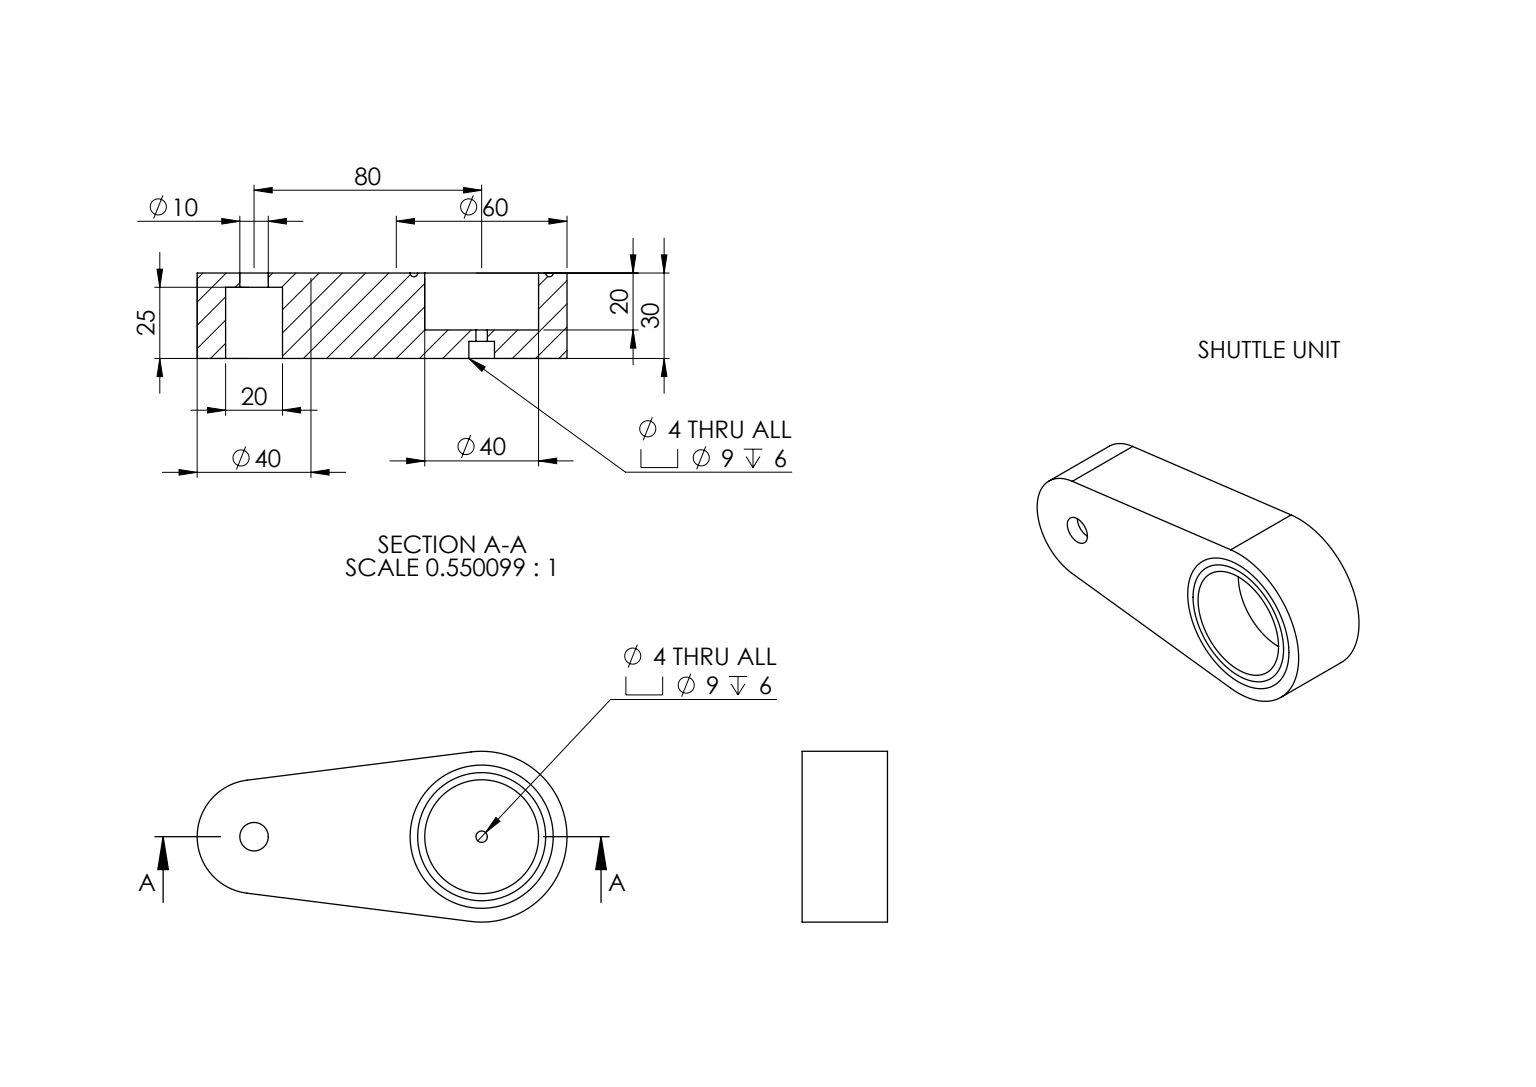
ISO-10303-21;
HEADER;
FILE_DESCRIPTION (('STEP AP214'),
    '1' );
FILE_NAME ('shuttle unit.step',
    '2026-10-24T08:20:21',
    ( '' ),
    ( '' ),
    'SwSTEP 2.0',
    'SolidWorks 2026',
    '' );
FILE_SCHEMA (( 'AUTOMOTIVE_DESIGN' ));
ENDSEC;

DATA;
#22=CARTESIAN_POINT ( 'NONE',  ( 0.000000000000000000, 0.000000000000000000, -30.00000000000000000 ) ) ;
#26=EDGE_CURVE ( 'NONE', #192, #3050, #3399, .T. ) ;
#35=CIRCLE ( 'NONE', #2208, 22.50000000000000355 ) ;
#36=ORIENTED_EDGE ( 'NONE', *, *, #1121, .F. ) ;
#52=VERTEX_POINT ( 'NONE', #3188 ) ;
#58=DIRECTION ( 'NONE',  ( 0.1250000000000000833, 0.9921567416492215186, -0.000000000000000000 ) ) ;
#59=DIRECTION ( 'NONE',  ( 1.000000000000000000, 0.000000000000000000, 0.000000000000000000 ) ) ;
#64=DIRECTION ( 'NONE',  ( -1.000000000000000000, 0.000000000000000000, 0.000000000000000000 ) ) ;
#70=DIRECTION ( 'NONE',  ( -1.000000000000000000, 0.000000000000000000, 0.000000000000000000 ) ) ;
#74=TOROIDAL_SURFACE ( 'NONE', #3494, 23.82500000000000284, 1.324999999999999956 ) ;
#77=DIRECTION ( 'NONE',  ( -1.000000000000000000, 0.000000000000000000, 0.000000000000000000 ) ) ;
#85=CARTESIAN_POINT ( 'NONE',  ( 0.000000000000000000, 0.000000000000000000, -30.00000000000000000 ) ) ;
#87=CARTESIAN_POINT ( 'NONE',  ( 0.000000000000000000, 0.000000000000000000, 0.000000000000000000 ) ) ;
#88=VECTOR ( 'NONE', #755, 999.9999999999998863 ) ;
#101=CARTESIAN_POINT ( 'NONE',  ( -85.00000000000000000, 0.000000000000000000, 0.001000000000000132727 ) ) ;
#103=CARTESIAN_POINT ( 'NONE',  ( -90.00000000000000000, 0.000000000000000000, -4.999999999999997335 ) ) ;
#107=CARTESIAN_POINT ( 'NONE',  ( -82.50000000000000000, -19.84313483298442904, 0.000000000000000000 ) ) ;
#115=ORIENTED_EDGE ( 'NONE', *, *, #3737, .T. ) ;
#116=PLANE ( 'NONE',  #1634 ) ;
#128=CARTESIAN_POINT ( 'NONE',  ( -80.00000000000000000, 0.000000000000000000, -30.00000000000000000 ) ) ;
#141=VECTOR ( 'NONE', #617, 1000.000000000000000 ) ;
#142=FACE_OUTER_BOUND ( 'NONE', #2988, .T. ) ;
#143=VERTEX_POINT ( 'NONE', #2588 ) ;
#159=SHAPE_REPRESENTATION ( 'shuttle unit', ( #2207 ), #968 ) ;
#161=EDGE_LOOP ( 'NONE', ( #2165, #1220, #1169, #2717, #1654 ) ) ;
#162=EDGE_CURVE ( 'NONE', #3091, #1782, #1381, .T. ) ;
#164=EDGE_CURVE ( 'NONE', #494, #1780, #3780, .T. ) ;
#166=CARTESIAN_POINT ( 'NONE',  ( 20.00000000000000000, 0.000000000000000000, 0.000000000000000000 ) ) ;
#178=ORIENTED_EDGE ( 'NONE', *, *, #1295, .F. ) ;
#179=CARTESIAN_POINT ( 'NONE',  ( -80.00000000000000000, 0.000000000000000000, 0.001000000000000132727 ) ) ;
#180=ORIENTED_EDGE ( 'NONE', *, *, #2925, .T. ) ;
#186=ORIENTED_EDGE ( 'NONE', *, *, #1295, .T. ) ;
#190=DIRECTION ( 'NONE',  ( -0.000000000000000000, 0.000000000000000000, 1.000000000000000000 ) ) ;
#192=VERTEX_POINT ( 'NONE', #3809 ) ;
#207=AXIS2_PLACEMENT_3D ( 'NONE', #2463, #2835, #972 ) ;
#215=CIRCLE ( 'NONE', #1581, 4.500000000000000888 ) ;
#223=ORIENTED_EDGE ( 'NONE', *, *, #2872, .T. ) ;
#233=SURFACE_SIDE_STYLE ('',( #1990 ) ) ;
#242=EDGE_LOOP ( 'NONE', ( #1908, #2671, #1653, #2183 ) ) ;
#255=DIRECTION ( 'NONE',  ( 0.000000000000000000, 0.000000000000000000, 1.000000000000000000 ) ) ;
#256=CYLINDRICAL_SURFACE ( 'NONE', #2880, 20.00000000000000000 ) ;
#261=VERTEX_POINT ( 'NONE', #657 ) ;
#273=AXIS2_PLACEMENT_3D ( 'NONE', #2448, #3041, #3118 ) ;
#276=VERTEX_POINT ( 'NONE', #1202 ) ;
#285=DIRECTION ( 'NONE',  ( -1.000000000000000000, 0.000000000000000000, 0.000000000000000000 ) ) ;
#296=CARTESIAN_POINT ( 'NONE',  ( 23.18826319173439288, -9.737913028511604452, 0.000000000000000000 ) ) ;
#301=ORIENTED_EDGE ( 'NONE', *, *, #2925, .F. ) ;
#302=FACE_OUTER_BOUND ( 'NONE', #2329, .T. ) ;
#304=EDGE_CURVE ( 'NONE', #2072, #2934, #2995, .T. ) ;
#307=ORIENTED_EDGE ( 'NONE', *, *, #1137, .F. ) ;
#321=CARTESIAN_POINT ( 'NONE',  ( 0.000000000000000000, 0.000000000000000000, -30.00000000000000000 ) ) ;
#326=ORIENTED_EDGE ( 'NONE', *, *, #2063, .T. ) ;
#328=VERTEX_POINT ( 'NONE', #1471 ) ;
#332=AXIS2_PLACEMENT_3D ( 'NONE', #2007, #2609, #441 ) ;
#346=PLANE ( 'NONE',  #504 ) ;
#349=CARTESIAN_POINT ( 'NONE',  ( 0.000000000000000000, 0.000000000000000000, -30.00000000000000000 ) ) ;
#355=VERTEX_POINT ( 'NONE', #1451 ) ;
#361=ADVANCED_FACE ( 'NONE', ( #2704, #2412, #2101 ), #1506, .T. ) ;
#363=DIRECTION ( 'NONE',  ( -1.000000000000000000, 0.000000000000000000, 0.000000000000000000 ) ) ;
#369=DIRECTION ( 'NONE',  ( -1.000000000000000000, 0.000000000000000000, 0.000000000000000000 ) ) ;
#372=DIRECTION ( 'NONE',  ( -0.9921567416492215186, 0.1250000000000000833, 0.000000000000000000 ) ) ;
#375=CARTESIAN_POINT ( 'NONE',  ( 0.000000000000000000, 0.000000000000000000, -30.00000000000000000 ) ) ;
#377=CIRCLE ( 'NONE', #827, 5.000000000000004441 ) ;
#379=CIRCLE ( 'NONE', #1823, 9.999999999999994671 ) ;
#381=DIRECTION ( 'NONE',  ( -0.000000000000000000, 0.000000000000000000, 1.000000000000000000 ) ) ;
#385=VERTEX_POINT ( 'NONE', #3241 ) ;
#389=ADVANCED_FACE ( 'NONE', ( #2979, #1826 ), #580, .T. ) ;
#390=CARTESIAN_POINT ( 'NONE',  ( 0.000000000000000000, 0.000000000000000000, -20.00000000000000000 ) ) ;
#394=DIRECTION ( 'NONE',  ( -0.3871933609746165406, -0.9219985364506716463, 2.410490433790582225E-18 ) ) ;
#397=VECTOR ( 'NONE', #716, 1000.000000000000000 ) ;
#406=ORIENTED_EDGE ( 'NONE', *, *, #3273, .T. ) ;
#411=ORIENTED_EDGE ( 'NONE', *, *, #905, .T. ) ;
#425=FACE_OUTER_BOUND ( 'NONE', #911, .T. ) ;
#434=DIRECTION ( 'NONE',  ( -0.000000000000000000, -0.000000000000000000, 1.000000000000000000 ) ) ;
#441=DIRECTION ( 'NONE',  ( 1.000000000000000000, 0.000000000000000000, 0.000000000000000000 ) ) ;
#443=AXIS2_PLACEMENT_3D ( 'NONE', #885, #2071, #3254 ) ;
#446=FACE_OUTER_BOUND ( 'NONE', #1984, .T. ) ;
#452=DIRECTION ( 'NONE',  ( -1.000000000000000000, 0.000000000000000000, 0.000000000000000000 ) ) ;
#454=FACE_OUTER_BOUND ( 'NONE', #746, .T. ) ;
#464=UNCERTAINTY_MEASURE_WITH_UNIT (LENGTH_MEASURE( 1.000000000000000082E-05 ), #2003, 'distance_accuracy_value', 'NONE');
#493=DIRECTION ( 'NONE',  ( 1.000000000000000000, 0.000000000000000000, 0.000000000000000000 ) ) ;
#494=VERTEX_POINT ( 'NONE', #975 ) ;
#495=DIRECTION ( 'NONE',  ( -0.000000000000000000, -0.000000000000000000, -1.000000000000000000 ) ) ;
#501=CARTESIAN_POINT ( 'NONE',  ( 0.000000000000000000, -0.000000000000000000, 0.000000000000000000 ) ) ;
#504=AXIS2_PLACEMENT_3D ( 'NONE', #2399, #1248, #996 ) ;
#515=DIRECTION ( 'NONE',  ( 0.000000000000000000, -1.000000000000000000, 0.000000000000000000 ) ) ;
#516=EDGE_CURVE ( 'NONE', #3615, #1351, #3346, .T. ) ;
#517=EDGE_CURVE ( 'NONE', #1737, #494, #1548, .T. ) ;
#528=AXIS2_PLACEMENT_3D ( 'NONE', #2164, #3336, #2490 ) ;
#530=DIRECTION ( 'NONE',  ( -1.000000000000000000, 0.000000000000000000, -0.000000000000000000 ) ) ;
#531=EDGE_LOOP ( 'NONE', ( #830, #1241, #942, #1732 ) ) ;
#540=DIRECTION ( 'NONE',  ( -0.000000000000000000, -0.000000000000000000, -1.000000000000000000 ) ) ;
#546=EDGE_CURVE ( 'NONE', #671, #2369, #590, .T. ) ;
#550=ORIENTED_EDGE ( 'NONE', *, *, #2872, .F. ) ;
#553=DIRECTION ( 'NONE',  ( 0.000000000000000000, -1.000000000000000000, 0.000000000000000000 ) ) ;
#563=EDGE_LOOP ( 'NONE', ( #2991, #2903, #3738, #178 ) ) ;
#566=EDGE_CURVE ( 'NONE', #3824, #3666, #844, .T. ) ;
#573=VERTEX_POINT ( 'NONE', #1808 ) ;
#575=FACE_BOUND ( 'NONE', #2885, .T. ) ;
#576=( GEOMETRIC_REPRESENTATION_CONTEXT ( 3 ) GLOBAL_UNCERTAINTY_ASSIGNED_CONTEXT ( ( #464 ) ) GLOBAL_UNIT_ASSIGNED_CONTEXT ( ( #2003, #2025, #3522 ) ) REPRESENTATION_CONTEXT ( 'NONE', 'WORKASPACE' ) );
#580=PLANE ( 'NONE',  #2653 ) ;
#581=CARTESIAN_POINT ( 'NONE',  ( 0.000000000000000000, -0.000000000000000000, 0.000000000000000000 ) ) ;
#590=CIRCLE ( 'NONE', #2764, 1.325000000000000622 ) ;
#593=CIRCLE ( 'NONE', #2088, 4.500000000000000888 ) ;
#595=CARTESIAN_POINT ( 'NONE',  ( -80.00000000000000000, 0.000000000000000000, -4.999999999999997335 ) ) ;
#598=AXIS2_PLACEMENT_3D ( 'NONE', #3513, #255, #2913 ) ;
#610=ORIENTED_EDGE ( 'NONE', *, *, #809, .F. ) ;
#617=DIRECTION ( 'NONE',  ( -0.000000000000000000, -0.000000000000000000, -1.000000000000000000 ) ) ;
#622=FACE_OUTER_BOUND ( 'NONE', #2781, .T. ) ;
#630=ORIENTED_EDGE ( 'NONE', *, *, #750, .T. ) ;
#641=DIRECTION ( 'NONE',  ( -0.9921567416492214075, 0.1250000000000000555, 0.000000000000000000 ) ) ;
#652=DIRECTION ( 'NONE',  ( 1.000000000000000000, 0.000000000000000000, 0.000000000000000000 ) ) ;
#655=EDGE_LOOP ( 'NONE', ( #3357, #2286, #1960, #1641, #907, #1356, #3483, #1912 ) ) ;
#657=CARTESIAN_POINT ( 'NONE',  ( -90.00000000000000000, 0.000000000000000000, -30.00000000000000000 ) ) ;
#662=CARTESIAN_POINT ( 'NONE',  ( -80.00000000000000000, 0.000000000000000000, -30.00000000000000000 ) ) ;
#665=EDGE_CURVE ( 'NONE', #3091, #3418, #215, .T. ) ;
#668=DIRECTION ( 'NONE',  ( -0.000000000000000000, -0.000000000000000000, -1.000000000000000000 ) ) ;
#671=VERTEX_POINT ( 'NONE', #3621 ) ;
#675=CARTESIAN_POINT ( 'NONE',  ( -3.750000000000001776, -29.76470224947664178, -30.00000000000000000 ) ) ;
#678=ADVANCED_FACE ( 'NONE', ( #302 ), #2688, .F. ) ;
#696=AXIS2_PLACEMENT_3D ( 'NONE', #375, #3331, #59 ) ;
#697=CARTESIAN_POINT ( 'NONE',  ( 0.000000000000000000, 0.000000000000000000, 0.000000000000000000 ) ) ;
#699=DIRECTION ( 'NONE',  ( 1.000000000000000000, 0.000000000000000000, 0.000000000000000000 ) ) ;
#707=EDGE_CURVE ( 'NONE', #1234, #1780, #2652, .T. ) ;
#716=DIRECTION ( 'NONE',  ( -0.000000000000000000, -1.000000000000000000, -0.000000000000000000 ) ) ;
#724=DIRECTION ( 'NONE',  ( 1.000000000000000000, 0.000000000000000000, 0.000000000000000000 ) ) ;
#731=CARTESIAN_POINT ( 'NONE',  ( 0.000000000000000000, 0.000000000000000000, 0.000000000000000000 ) ) ;
#732=ORIENTED_EDGE ( 'NONE', *, *, #3728, .T. ) ;
#740=EDGE_CURVE ( 'NONE', #1954, #1234, #2219, .T. ) ;
#746=EDGE_LOOP ( 'NONE', ( #610, #2576 ) ) ;
#750=EDGE_CURVE ( 'NONE', #2723, #2369, #1277, .T. ) ;
#755=DIRECTION ( 'NONE',  ( 0.9921567416492215186, 0.1250000000000001665, 0.000000000000000000 ) ) ;
#757=VERTEX_POINT ( 'NONE', #1550 ) ;
#758=VERTEX_POINT ( 'NONE', #107 ) ;
#764=AXIS2_PLACEMENT_3D ( 'NONE', #179, #3725, #2829 ) ;
#769=PLANE ( 'NONE',  #2386 ) ;
#791=ADVANCED_BREP_SHAPE_REPRESENTATION ( '', ( #1966, #2207 ), #968 ) ;
#792=DIRECTION ( 'NONE',  ( 0.000000000000000000, 0.000000000000000000, 1.000000000000000000 ) ) ;
#803=DIRECTION ( 'NONE',  ( 1.000000000000000000, 0.000000000000000000, 0.000000000000000000 ) ) ;
#809=EDGE_CURVE ( 'NONE', #385, #671, #35, .T. ) ;
#813=CYLINDRICAL_SURFACE ( 'NONE', #1460, 4.499999999999997335 ) ;
#820=CARTESIAN_POINT ( 'NONE',  ( 0.000000000000000000, 0.000000000000000000, 0.000000000000000000 ) ) ;
#826=CIRCLE ( 'NONE', #1320, 20.00000000000000355 ) ;
#827=AXIS2_PLACEMENT_3D ( 'NONE', #1745, #2304, #2589 ) ;
#830=ORIENTED_EDGE ( 'NONE', *, *, #809, .T. ) ;
#838=CARTESIAN_POINT ( 'NONE',  ( 0.000000000000000000, 0.000000000000000000, -30.00000000000000000 ) ) ;
#844=CIRCLE ( 'NONE', #3019, 30.00000000000000000 ) ;
#849=CYLINDRICAL_SURFACE ( 'NONE', #764, 5.000000000000004441 ) ;
#850=ORIENTED_EDGE ( 'NONE', *, *, #2359, .T. ) ;
#852=ORIENTED_EDGE ( 'NONE', *, *, #1811, .T. ) ;
#853=PRODUCT_DEFINITION_FORMATION_WITH_SPECIFIED_SOURCE ( 'ANY', '', #3643, .NOT_KNOWN. ) ;
#854=EDGE_CURVE ( 'NONE', #3666, #1351, #1907, .T. ) ;
#858=LINE ( 'NONE', #2300, #1159 ) ;
#862=ORIENTED_EDGE ( 'NONE', *, *, #1617, .F. ) ;
#885=CARTESIAN_POINT ( 'NONE',  ( 0.000000000000000000, 0.000000000000000000, 0.000000000000000000 ) ) ;
#887=CIRCLE ( 'NONE', #2621, 5.000000000000004441 ) ;
#891=CARTESIAN_POINT ( 'NONE',  ( 0.000000000000000000, 0.000000000000000000, -30.00000000000000000 ) ) ;
#894=AXIS2_PLACEMENT_3D ( 'NONE', #2296, #1423, #1955 ) ;
#900=VECTOR ( 'NONE', #3282, 1000.000000000000000 ) ;
#905=EDGE_CURVE ( 'NONE', #1737, #2422, #2837, .T. ) ;
#907=ORIENTED_EDGE ( 'NONE', *, *, #566, .F. ) ;
#911=EDGE_LOOP ( 'NONE', ( #1275, #2494 ) ) ;
#914=LINE ( 'NONE', #2097, #900 ) ;
#918=CARTESIAN_POINT ( 'NONE',  ( 20.00000000000000000, 0.000000000000000000, -20.00000000000000000 ) ) ;
#927=ORIENTED_EDGE ( 'NONE', *, *, #3644, .T. ) ;
#937=ADVANCED_FACE ( 'NONE', ( #3402, #454 ), #2465, .T. ) ;
#938=DIRECTION ( 'NONE',  ( 1.000000000000000000, 0.000000000000000000, 0.000000000000000000 ) ) ;
#942=ORIENTED_EDGE ( 'NONE', *, *, #3532, .T. ) ;
#943=EDGE_CURVE ( 'NONE', #1799, #2993, #2254, .T. ) ;
#945=LINE ( 'NONE', #2951, #1884 ) ;
#952=AXIS2_PLACEMENT_3D ( 'NONE', #2980, #2082, #70 ) ;
#962=DIRECTION ( 'NONE',  ( 0.000000000000000000, 0.000000000000000000, 1.000000000000000000 ) ) ;
#963=DIRECTION ( 'NONE',  ( -1.000000000000000000, 0.000000000000000000, 0.000000000000000000 ) ) ;
#968=( GEOMETRIC_REPRESENTATION_CONTEXT ( 3 ) GLOBAL_UNCERTAINTY_ASSIGNED_CONTEXT ( ( #3201 ) ) GLOBAL_UNIT_ASSIGNED_CONTEXT ( ( #2883, #3143, #1928 ) ) REPRESENTATION_CONTEXT ( 'NONE', 'WORKASPACE' ) );
#971=VECTOR ( 'NONE', #1427, 1000.000000000000114 ) ;
#972=DIRECTION ( 'NONE',  ( -1.000000000000000000, 0.000000000000000000, 0.000000000000000000 ) ) ;
#975=CARTESIAN_POINT ( 'NONE',  ( -70.00000000000000000, -21.41798680385620202, -30.00000000000000000 ) ) ;
#977=EDGE_CURVE ( 'NONE', #3418, #3091, #593, .T. ) ;
#991=DIRECTION ( 'NONE',  ( -0.000000000000000000, -0.000000000000000000, -1.000000000000000000 ) ) ;
#996=DIRECTION ( 'NONE',  ( -0.000000000000000000, 0.000000000000000000, 1.000000000000000000 ) ) ;
#999=DIRECTION ( 'NONE',  ( -0.000000000000000000, -0.000000000000000000, -1.000000000000000000 ) ) ;
#1003=VERTEX_POINT ( 'NONE', #3667 ) ;
#1008=CARTESIAN_POINT ( 'NONE',  ( -3.750000000000001776, -29.76470224947664178, -4.999999999999997335 ) ) ;
#1009=EDGE_CURVE ( 'NONE', #1780, #573, #3113, .T. ) ;
#1014=ORIENTED_EDGE ( 'NONE', *, *, #665, .F. ) ;
#1021=DIRECTION ( 'NONE',  ( 0.3871933609746164295, 0.9219985364506716463, -2.410490433790583766E-18 ) ) ;
#1024=EDGE_LOOP ( 'NONE', ( #862, #732, #2751, #550 ) ) ;
#1031=DIRECTION ( 'NONE',  ( -1.000000000000000000, 0.000000000000000000, 0.000000000000000000 ) ) ;
#1037=DIRECTION ( 'NONE',  ( 1.000000000000000000, 0.000000000000000000, 0.000000000000000000 ) ) ;
#1063=ORIENTED_EDGE ( 'NONE', *, *, #164, .T. ) ;
#1068=VERTEX_POINT ( 'NONE', #2932 ) ;
#1077=AXIS2_PLACEMENT_3D ( 'NONE', #128, #1951, #1325 ) ;
#1080=AXIS2_PLACEMENT_3D ( 'NONE', #3179, #530, #2863 ) ;
#1090=FACE_OUTER_BOUND ( 'NONE', #2921, .T. ) ;
#1094=EDGE_LOOP ( 'NONE', ( #1195, #2367 ) ) ;
#1101=CIRCLE ( 'NONE', #1965, 2.000000000000001776 ) ;
#1102=CARTESIAN_POINT ( 'NONE',  ( 0.000000000000000000, 0.000000000000000000, 0.000000000000000000 ) ) ;
#1109=ORIENTED_EDGE ( 'NONE', *, *, #1617, .T. ) ;
#1111=CARTESIAN_POINT ( 'NONE',  ( 2.000000000000001776, 0.000000000000000000, -24.00000000000000000 ) ) ;
#1114=DIRECTION ( 'NONE',  ( 0.000000000000000000, 0.000000000000000000, 1.000000000000000000 ) ) ;
#1120=EDGE_LOOP ( 'NONE', ( #2830, #326, #2091, #1837 ) ) ;
#1121=EDGE_CURVE ( 'NONE', #1151, #3615, #1672, .T. ) ;
#1124=CARTESIAN_POINT ( 'NONE',  ( -82.50000000000000000, 19.84313483298442193, -30.00000000000000000 ) ) ;
#1125=DIRECTION ( 'NONE',  ( -1.000000000000000000, 0.000000000000000000, 0.000000000000000000 ) ) ;
#1126=EDGE_CURVE ( 'NONE', #355, #2934, #3519, .T. ) ;
#1127=ORIENTED_EDGE ( 'NONE', *, *, #1126, .F. ) ;
#1133=EDGE_CURVE ( 'NONE', #1954, #494, #858, .T. ) ;
#1137=EDGE_CURVE ( 'NONE', #143, #1068, #1101, .T. ) ;
#1140=ADVANCED_FACE ( 'NONE', ( #1090 ), #813, .F. ) ;
#1151=VERTEX_POINT ( 'NONE', #3205 ) ;
#1159=VECTOR ( 'NONE', #553, 1000.000000000000000 ) ;
#1160=ORIENTED_EDGE ( 'NONE', *, *, #3532, .F. ) ;
#1169=ORIENTED_EDGE ( 'NONE', *, *, #707, .T. ) ;
#1174=ORIENTED_EDGE ( 'NONE', *, *, #3728, .F. ) ;
#1185=CARTESIAN_POINT ( 'NONE',  ( -80.00000000000000000, 0.000000000000000000, -4.999999999999997335 ) ) ;
#1192=TOROIDAL_SURFACE ( 'NONE', #1316, 23.82500000000000284, 1.324999999999999956 ) ;
#1194=DIRECTION ( 'NONE',  ( -0.000000000000000000, -0.000000000000000000, 1.000000000000000000 ) ) ;
#1195=ORIENTED_EDGE ( 'NONE', *, *, #1897, .F. ) ;
#1199=AXIS2_PLACEMENT_3D ( 'NONE', #1111, #2352, #2642 ) ;
#1202=CARTESIAN_POINT ( 'NONE',  ( -90.00000000000000000, -17.32050807568877815, -30.00000000000000000 ) ) ;
#1213=EDGE_CURVE ( 'NONE', #573, #758, #3350, .T. ) ;
#1217=AXIS2_PLACEMENT_3D ( 'NONE', #349, #2733, #963 ) ;
#1220=ORIENTED_EDGE ( 'NONE', *, *, #2326, .F. ) ;
#1233=DIRECTION ( 'NONE',  ( 1.000000000000000000, 0.000000000000000000, 0.000000000000000000 ) ) ;
#1234=VERTEX_POINT ( 'NONE', #1537 ) ;
#1241=ORIENTED_EDGE ( 'NONE', *, *, #546, .T. ) ;
#1248=DIRECTION ( 'NONE',  ( -1.000000000000000000, 0.000000000000000000, -0.000000000000000000 ) ) ;
#1275=ORIENTED_EDGE ( 'NONE', *, *, #3443, .T. ) ;
#1277=CIRCLE ( 'NONE', #273, 25.15000000000000213 ) ;
#1282=CARTESIAN_POINT ( 'NONE',  ( -3.749999999999998224, -29.76470224947664533, -30.00000000000000000 ) ) ;
#1284=EDGE_CURVE ( 'NONE', #261, #1954, #1523, .T. ) ;
#1286=CARTESIAN_POINT ( 'NONE',  ( -70.00000000000000000, 0.000000000000000000, -4.999999999999997335 ) ) ;
#1289=CARTESIAN_POINT ( 'NONE',  ( 0.000000000000000000, 0.000000000000000000, -30.00000000000000000 ) ) ;
#1295=EDGE_CURVE ( 'NONE', #2309, #1351, #2897, .T. ) ;
#1298=CARTESIAN_POINT ( 'NONE',  ( 0.000000000000000000, 0.000000000000000000, -24.00000000000000000 ) ) ;
#1310=LINE ( 'NONE', #2206, #1706 ) ;
#1311=LINE ( 'NONE', #101, #2818 ) ;
#1316=AXIS2_PLACEMENT_3D ( 'NONE', #501, #3743, #2848 ) ;
#1317=DIRECTION ( 'NONE',  ( 0.000000000000000000, 0.000000000000000000, 1.000000000000000000 ) ) ;
#1320=AXIS2_PLACEMENT_3D ( 'NONE', #595, #1194, #3572 ) ;
#1323=CIRCLE ( 'NONE', #1633, 4.499999999999993783 ) ;
#1325=DIRECTION ( 'NONE',  ( 1.000000000000000000, 0.000000000000000000, 0.000000000000000000 ) ) ;
#1331=DIRECTION ( 'NONE',  ( -0.9921567416492215186, 0.1250000000000000833, 0.000000000000000000 ) ) ;
#1332=FACE_OUTER_BOUND ( 'NONE', #2931, .T. ) ;
#1336=VECTOR ( 'NONE', #999, 1000.000000000000000 ) ;
#1342=CARTESIAN_POINT ( 'NONE',  ( 0.000000000000000000, 0.000000000000000000, -20.00000000000000000 ) ) ;
#1351=VERTEX_POINT ( 'NONE', #2801 ) ;
#1352=LINE ( 'NONE', #1992, #2194 ) ;
#1354=CARTESIAN_POINT ( 'NONE',  ( -3.750000000000004441, 29.76470224947664533, -30.00000000000000000 ) ) ;
#1356=ORIENTED_EDGE ( 'NONE', *, *, #2359, .F. ) ;
#1363=LINE ( 'NONE', #1608, #3303 ) ;
#1365=CYLINDRICAL_SURFACE ( 'NONE', #1077, 20.00000000000000355 ) ;
#1375=APPLICATION_CONTEXT ( 'automotive_design' ) ;
#1377=DIRECTION ( 'NONE',  ( -0.000000000000000000, -0.000000000000000000, 1.000000000000000000 ) ) ;
#1380=EDGE_LOOP ( 'NONE', ( #3293, #2842 ) ) ;
#1381=LINE ( 'NONE', #1715, #1407 ) ;
#1398=ORIENTED_EDGE ( 'NONE', *, *, #2612, .T. ) ;
#1406=ADVANCED_FACE ( 'NONE', ( #2861 ), #1192, .F. ) ;
#1407=VECTOR ( 'NONE', #540, 1000.000000000000000 ) ;
#1412=ORIENTED_EDGE ( 'NONE', *, *, #1811, .F. ) ;
#1423=DIRECTION ( 'NONE',  ( -0.000000000000000000, 0.000000000000000000, 1.000000000000000000 ) ) ;
#1427=DIRECTION ( 'NONE',  ( -0.9921567416492214075, 0.1250000000000000555, 0.000000000000000000 ) ) ;
#1428=CARTESIAN_POINT ( 'NONE',  ( -80.00000000000000000, 0.000000000000000000, -4.999999999999997335 ) ) ;
#1431=DIRECTION ( 'NONE',  ( -1.795453617517838654E-17, 1.015442787603507153E-17, 1.000000000000000000 ) ) ;
#1436=ADVANCED_FACE ( 'NONE', ( #3107 ), #1365, .T. ) ;
#1441=AXIS2_PLACEMENT_3D ( 'NONE', #891, #2663, #652 ) ;
#1445=DIRECTION ( 'NONE',  ( -0.000000000000000000, -0.000000000000000000, -1.000000000000000000 ) ) ;
#1447=CARTESIAN_POINT ( 'NONE',  ( -90.00000000000000000, 0.000000000000000000, -30.00000000000000000 ) ) ;
#1451=CARTESIAN_POINT ( 'NONE',  ( -20.00000000000000000, 2.449293598294706513E-15, 0.000000000000000000 ) ) ;
#1460=AXIS2_PLACEMENT_3D ( 'NONE', #1741, #1445, #2314 ) ;
#1462=ORIENTED_EDGE ( 'NONE', *, *, #750, .F. ) ;
#1467=CARTESIAN_POINT ( 'NONE',  ( -80.00000000000000000, 0.000000000000000000, -30.00000000000000000 ) ) ;
#1469=ORIENTED_EDGE ( 'NONE', *, *, #516, .T. ) ;
#1471=CARTESIAN_POINT ( 'NONE',  ( -20.00000000000000000, 2.449293598294706513E-15, -20.00000000000000000 ) ) ;
#1490=ORIENTED_EDGE ( 'NONE', *, *, #3224, .T. ) ;
#1491=DIRECTION ( 'NONE',  ( -1.000000000000000000, 0.000000000000000000, 0.000000000000000000 ) ) ;
#1496=AXIS2_PLACEMENT_3D ( 'NONE', #321, #1969, #724 ) ;
#1506=PLANE ( 'NONE',  #3764 ) ;
#1523=CIRCLE ( 'NONE', #1899, 9.999999999999994671 ) ;
#1534=PLANE ( 'NONE',  #696 ) ;
#1537=CARTESIAN_POINT ( 'NONE',  ( -70.00000000000000000, 0.000000000000000000, -4.999999999999997335 ) ) ;
#1548=LINE ( 'NONE', #675, #2274 ) ;
#1550=CARTESIAN_POINT ( 'NONE',  ( -85.00000000000000000, 0.000000000000000000, -4.999999999999997335 ) ) ;
#1557=ORIENTED_EDGE ( 'NONE', *, *, #740, .T. ) ;
#1558=DIRECTION ( 'NONE',  ( 0.1250000000000001665, -0.9921567416492215186, 0.000000000000000000 ) ) ;
#1562=DIRECTION ( 'NONE',  ( -0.000000000000000000, 0.000000000000000000, 1.000000000000000000 ) ) ;
#1564=STYLED_ITEM('',(#3860),#1966);
#1581=AXIS2_PLACEMENT_3D ( 'NONE', #2728, #2672, #1491 ) ;
#1591=DIRECTION ( 'NONE',  ( 0.000000000000000000, -0.000000000000000000, -1.000000000000000000 ) ) ;
#1595=FACE_OUTER_BOUND ( 'NONE', #1801, .T. ) ;
#1603=CARTESIAN_POINT ( 'NONE',  ( -3.750000000000004441, 29.76470224947664533, 0.000000000000000000 ) ) ;
#1608=CARTESIAN_POINT ( 'NONE',  ( -20.00000000000000000, 2.449293598294706513E-15, -20.00000000000000000 ) ) ;
#1617=EDGE_CURVE ( 'NONE', #1003, #2788, #3746, .T. ) ;
#1621=ORIENTED_EDGE ( 'NONE', *, *, #2989, .T. ) ;
#1633=AXIS2_PLACEMENT_3D ( 'NONE', #1289, #668, #77 ) ;
#1634=AXIS2_PLACEMENT_3D ( 'NONE', #1354, #1558, #1891 ) ;
#1641=ORIENTED_EDGE ( 'NONE', *, *, #1820, .T. ) ;
#1644=DIRECTION ( 'NONE',  ( -0.000000000000000000, -0.000000000000000000, -1.000000000000000000 ) ) ;
#1653=ORIENTED_EDGE ( 'NONE', *, *, #2499, .T. ) ;
#1654=ORIENTED_EDGE ( 'NONE', *, *, #3224, .F. ) ;
#1663=ADVANCED_FACE ( 'NONE', ( #2470, #3656 ), #1534, .F. ) ;
#1667=ADVANCED_FACE ( 'NONE', ( #3289 ), #346, .F. ) ;
#1672=LINE ( 'NONE', #1124, #2834 ) ;
#1675=CARTESIAN_POINT ( 'NONE',  ( -70.00000000000000000, -21.41798680385620202, -30.00000000000000000 ) ) ;
#1682=PLANE ( 'NONE',  #1080 ) ;
#1686=CARTESIAN_POINT ( 'NONE',  ( 4.500000000000000000, 5.510910596163089556E-16, -24.00000000000000000 ) ) ;
#1687=EDGE_LOOP ( 'NONE', ( #2677, #3663 ) ) ;
#1691=ORIENTED_EDGE ( 'NONE', *, *, #740, .F. ) ;
#1693=FACE_OUTER_BOUND ( 'NONE', #2600, .T. ) ;
#1697=FILL_AREA_STYLE ('',( #1952 ) ) ;
#1700=AXIS2_PLACEMENT_3D ( 'NONE', #3794, #3175, #1731 ) ;
#1706=VECTOR ( 'NONE', #1331, 999.9999999999998863 ) ;
#1711=FACE_OUTER_BOUND ( 'NONE', #1380, .T. ) ;
#1712=EDGE_CURVE ( 'NONE', #1151, #276, #3431, .T. ) ;
#1715=CARTESIAN_POINT ( 'NONE',  ( 4.499999999999997335, 5.510910596163085611E-16, -30.00000000000000000 ) ) ;
#1716=AXIS2_PLACEMENT_3D ( 'NONE', #2513, #381, #2144 ) ;
#1726=ORIENTED_EDGE ( 'NONE', *, *, #2799, .F. ) ;
#1731=DIRECTION ( 'NONE',  ( 1.000000000000000000, 0.000000000000000000, 0.000000000000000000 ) ) ;
#1732=ORIENTED_EDGE ( 'NONE', *, *, #3644, .F. ) ;
#1736=DIRECTION ( 'NONE',  ( -0.000000000000000000, -0.000000000000000000, -1.000000000000000000 ) ) ;
#1737=VERTEX_POINT ( 'NONE', #3043 ) ;
#1741=CARTESIAN_POINT ( 'NONE',  ( 0.000000000000000000, 0.000000000000000000, -30.00000000000000000 ) ) ;
#1743=ORIENTED_EDGE ( 'NONE', *, *, #2063, .F. ) ;
#1745=CARTESIAN_POINT ( 'NONE',  ( -80.00000000000000000, 0.000000000000000000, -4.999999999999997335 ) ) ;
#1746=ADVANCED_FACE ( 'NONE', ( #622 ), #3001, .T. ) ;
#1747=ORIENTED_EDGE ( 'NONE', *, *, #1712, .T. ) ;
#1750=SHAPE_REPRESENTATION_RELATIONSHIP ( 'NONE' , 'NONE' ,  #159, #791 ) ;
#1752=AXIS2_PLACEMENT_3D ( 'NONE', #662, #2161, #699 ) ;
#1764=CARTESIAN_POINT ( 'NONE',  ( 30.00000000000000000, 0.000000000000000000, 0.000000000000000000 ) ) ;
#1767=ORIENTED_EDGE ( 'NONE', *, *, #546, .F. ) ;
#1769=CARTESIAN_POINT ( 'NONE',  ( 0.000000000000000000, 0.000000000000000000, -4.999999999999997335 ) ) ;
#1770=DIRECTION ( 'NONE',  ( -0.9219985364506716463, 0.3871933609746164295, -2.048578313426146660E-17 ) ) ;
#1772=EDGE_LOOP ( 'NONE', ( #852, #1109 ) ) ;
#1777=EDGE_CURVE ( 'NONE', #328, #355, #1363, .T. ) ;
#1780=VERTEX_POINT ( 'NONE', #3158 ) ;
#1781=VECTOR ( 'NONE', #1114, 1000.000000000000000 ) ;
#1782=VERTEX_POINT ( 'NONE', #2487 ) ;
#1794=PRODUCT_DEFINITION ( 'UNKNOWN', '', #853, #2727 ) ;
#1799=VERTEX_POINT ( 'NONE', #1909 ) ;
#1801=EDGE_LOOP ( 'NONE', ( #1174, #1412, #223, #3437 ) ) ;
#1804=FACE_OUTER_BOUND ( 'NONE', #1120, .T. ) ;
#1808=CARTESIAN_POINT ( 'NONE',  ( -82.50000000000000000, -19.84313483298442904, -4.999999999999997335 ) ) ;
#1811=EDGE_CURVE ( 'NONE', #2788, #1003, #887, .T. ) ;
#1820=EDGE_CURVE ( 'NONE', #1151, #3666, #3673, .T. ) ;
#1823=AXIS2_PLACEMENT_3D ( 'NONE', #1428, #3237, #1125 ) ;
#1826=FACE_OUTER_BOUND ( 'NONE', #161, .T. ) ;
#1837=ORIENTED_EDGE ( 'NONE', *, *, #3556, .F. ) ;
#1850=CARTESIAN_POINT ( 'NONE',  ( -82.50000000000000000, -19.84313483298442904, -30.00000000000000000 ) ) ;
#1851=CARTESIAN_POINT ( 'NONE',  ( -80.00000000000000000, 0.000000000000000000, 0.001000000000000132727 ) ) ;
#1852=ORIENTED_EDGE ( 'NONE', *, *, #1133, .T. ) ;
#1869=EDGE_LOOP ( 'NONE', ( #2204, #2702, #2155, #2272 ) ) ;
#1870=CARTESIAN_POINT ( 'NONE',  ( 0.000000000000000000, 0.000000000000000000, -20.00000000000000000 ) ) ;
#1872=CYLINDRICAL_SURFACE ( 'NONE', #2700, 4.499999999999997335 ) ;
#1879=VECTOR ( 'NONE', #515, 1000.000000000000000 ) ;
#1882=CARTESIAN_POINT ( 'NONE',  ( -3.750000000000004441, 29.76470224947664533, -30.00000000000000000 ) ) ;
#1884=VECTOR ( 'NONE', #2349, 1000.000000000000000 ) ;
#1887=ADVANCED_FACE ( 'NONE', ( #2047 ), #2605, .F. ) ;
#1891=DIRECTION ( 'NONE',  ( 0.9921567416492214075, 0.1250000000000001388, 0.000000000000000000 ) ) ;
#1893=EDGE_CURVE ( 'NONE', #2934, #355, #3558, .T. ) ;
#1897=EDGE_CURVE ( 'NONE', #757, #2595, #377, .T. ) ;
#1899=AXIS2_PLACEMENT_3D ( 'NONE', #1467, #2662, #2417 ) ;
#1902=CARTESIAN_POINT ( 'NONE',  ( -3.749999999999998224, 29.76470224947664533, -30.00000000000000000 ) ) ;
#1907=LINE ( 'NONE', #1902, #2711 ) ;
#1908=ORIENTED_EDGE ( 'NONE', *, *, #3326, .T. ) ;
#1909=CARTESIAN_POINT ( 'NONE',  ( -90.00000000000000000, 0.000000000000000000, -4.999999999999997335 ) ) ;
#1912=ORIENTED_EDGE ( 'NONE', *, *, #1133, .F. ) ;
#1918=ORIENTED_EDGE ( 'NONE', *, *, #707, .F. ) ;
#1926=SHAPE_DEFINITION_REPRESENTATION ( #3429, #159 ) ;
#1928=( NAMED_UNIT ( * ) SI_UNIT ( $, .STERADIAN. ) SOLID_ANGLE_UNIT ( ) );
#1929=ADVANCED_FACE ( 'NONE', ( #1693 ), #74, .F. ) ;
#1935=DIRECTION ( 'NONE',  ( 0.000000000000000000, 0.000000000000000000, 1.000000000000000000 ) ) ;
#1940=MECHANICAL_DESIGN_GEOMETRIC_PRESENTATION_REPRESENTATION('',(#1564),#576);
#1948=PRODUCT_CONTEXT ( 'NONE', #2027, 'mechanical' ) ;
#1949=EDGE_CURVE ( 'NONE', #2595, #757, #3246, .T. ) ;
#1951=DIRECTION ( 'NONE',  ( 0.000000000000000000, 0.000000000000000000, 1.000000000000000000 ) ) ;
#1952=FILL_AREA_STYLE_COLOUR ( '', #2956 ) ;
#1954=VERTEX_POINT ( 'NONE', #2936 ) ;
#1955=DIRECTION ( 'NONE',  ( 1.000000000000000000, 0.000000000000000000, 0.000000000000000000 ) ) ;
#1960=ORIENTED_EDGE ( 'NONE', *, *, #1712, .F. ) ;
#1962=CIRCLE ( 'NONE', #1716, 30.00000000000000000 ) ;
#1965=AXIS2_PLACEMENT_3D ( 'NONE', #2563, #495, #3475 ) ;
#1966=MANIFOLD_SOLID_BREP ( 'CBORE for M4 Pan Head Screw1', #3341 ) ;
#1967=ORIENTED_EDGE ( 'NONE', *, *, #3796, .F. ) ;
#1969=DIRECTION ( 'NONE',  ( 0.000000000000000000, 0.000000000000000000, 1.000000000000000000 ) ) ;
#1974=PRESENTATION_STYLE_ASSIGNMENT (( #2268 ) ) ;
#1976=ORIENTED_EDGE ( 'NONE', *, *, #3737, .F. ) ;
#1977=DIRECTION ( 'NONE',  ( 1.000000000000000000, 0.000000000000000000, 0.000000000000000000 ) ) ;
#1979=CARTESIAN_POINT ( 'NONE',  ( 2.000000000000001776, 2.449293598294708880E-16, -20.00000000000000000 ) ) ;
#1984=EDGE_LOOP ( 'NONE', ( #1063, #1918, #1691, #1852 ) ) ;
#1986=DIRECTION ( 'NONE',  ( 0.000000000000000000, 0.000000000000000000, -1.000000000000000000 ) ) ;
#1988=ADVANCED_FACE ( 'NONE', ( #1804 ), #2996, .F. ) ;
#1990=SURFACE_STYLE_FILL_AREA ( #1697 ) ;
#1992=CARTESIAN_POINT ( 'NONE',  ( -90.00000000000000000, -17.32050807568877460, -30.00000000000000000 ) ) ;
#1993=ORIENTED_EDGE ( 'NONE', *, *, #3765, .F. ) ;
#2003=( LENGTH_UNIT ( ) NAMED_UNIT ( * ) SI_UNIT ( .MILLI., .METRE. ) );
#2007=CARTESIAN_POINT ( 'NONE',  ( 0.000000000000000000, 0.000000000000000000, -20.00000000000000000 ) ) ;
#2018=CARTESIAN_POINT ( 'NONE',  ( 0.000000000000000000, 0.000000000000000000, -20.00000000000000000 ) ) ;
#2025=( NAMED_UNIT ( * ) PLANE_ANGLE_UNIT ( ) SI_UNIT ( $, .RADIAN. ) );
#2027=APPLICATION_CONTEXT ( 'automotive_design' ) ;
#2035=FACE_OUTER_BOUND ( 'NONE', #1024, .T. ) ;
#2040=ORIENTED_EDGE ( 'NONE', *, *, #3678, .F. ) ;
#2041=DIRECTION ( 'NONE',  ( 0.000000000000000000, 0.000000000000000000, 1.000000000000000000 ) ) ;
#2043=DIRECTION ( 'NONE',  ( 1.000000000000000000, 0.000000000000000000, 0.000000000000000000 ) ) ;
#2047=FACE_OUTER_BOUND ( 'NONE', #3318, .T. ) ;
#2061=DIRECTION ( 'NONE',  ( -0.000000000000000000, -0.000000000000000000, -1.000000000000000000 ) ) ;
#2063=EDGE_CURVE ( 'NONE', #3050, #143, #3100, .T. ) ;
#2071=DIRECTION ( 'NONE',  ( -0.000000000000000000, 0.000000000000000000, 1.000000000000000000 ) ) ;
#2072=VERTEX_POINT ( 'NONE', #3135 ) ;
#2074=ORIENTED_EDGE ( 'NONE', *, *, #905, .F. ) ;
#2079=ORIENTED_EDGE ( 'NONE', *, *, #3159, .T. ) ;
#2081=DIRECTION ( 'NONE',  ( -0.000000000000000000, -0.000000000000000000, 1.000000000000000000 ) ) ;
#2082=DIRECTION ( 'NONE',  ( -0.000000000000000000, -0.000000000000000000, -1.000000000000000000 ) ) ;
#2088=AXIS2_PLACEMENT_3D ( 'NONE', #1298, #991, #1031 ) ;
#2091=ORIENTED_EDGE ( 'NONE', *, *, #1137, .T. ) ;
#2097=CARTESIAN_POINT ( 'NONE',  ( -90.00000000000000000, 0.000000000000000000, -30.00001199999999812 ) ) ;
#2101=FACE_BOUND ( 'NONE', #3292, .T. ) ;
#2121=CARTESIAN_POINT ( 'NONE',  ( -21.96661513093725659, 9.224881825220236919, 2.544523588129261943E-16 ) ) ;
#2129=CIRCLE ( 'NONE', #443, 25.15000000000000213 ) ;
#2134=CARTESIAN_POINT ( 'NONE',  ( -23.18826319173439288, 9.737913028511604452, 0.000000000000000000 ) ) ;
#2137=CIRCLE ( 'NONE', #3630, 2.000000000000001776 ) ;
#2144=DIRECTION ( 'NONE',  ( 1.000000000000000000, 0.000000000000000000, 0.000000000000000000 ) ) ;
#2155=ORIENTED_EDGE ( 'NONE', *, *, #304, .T. ) ;
#2159=AXIS2_PLACEMENT_3D ( 'NONE', #1342, #3139, #1037 ) ;
#2161=DIRECTION ( 'NONE',  ( -0.000000000000000000, 0.000000000000000000, 1.000000000000000000 ) ) ;
#2164=CARTESIAN_POINT ( 'NONE',  ( 0.000000000000000000, 0.000000000000000000, -20.00000000000000000 ) ) ;
#2165=ORIENTED_EDGE ( 'NONE', *, *, #943, .F. ) ;
#2183=ORIENTED_EDGE ( 'NONE', *, *, #943, .T. ) ;
#2184=ORIENTED_EDGE ( 'NONE', *, *, #2612, .F. ) ;
#2186=AXIS2_PLACEMENT_3D ( 'NONE', #2984, #3639, #938 ) ;
#2190=AXIS2_PLACEMENT_3D ( 'NONE', #3747, #792, #1977 ) ;
#2194=VECTOR ( 'NONE', #2908, 1000.000000000000000 ) ;
#2196=ORIENTED_EDGE ( 'NONE', *, *, #854, .F. ) ;
#2204=ORIENTED_EDGE ( 'NONE', *, *, #1777, .F. ) ;
#2206=CARTESIAN_POINT ( 'NONE',  ( -3.750000000000001776, -29.76470224947664178, 0.000000000000000000 ) ) ;
#2207=AXIS2_PLACEMENT_3D ( 'NONE', #820, #2246, #3194 ) ;
#2208=AXIS2_PLACEMENT_3D ( 'NONE', #697, #1591, #2762 ) ;
#2219=LINE ( 'NONE', #2819, #2894 ) ;
#2227=DIRECTION ( 'NONE',  ( 0.000000000000000000, -0.000000000000000000, -1.000000000000000000 ) ) ;
#2230=ADVANCED_FACE ( 'NONE', ( #2564 ), #256, .F. ) ;
#2231=EDGE_CURVE ( 'NONE', #261, #276, #3517, .T. ) ;
#2238=ADVANCED_FACE ( 'NONE', ( #575, #1711 ), #3777, .F. ) ;
#2246=DIRECTION ( 'NONE',  ( 0.000000000000000000, 0.000000000000000000, 1.000000000000000000 ) ) ;
#2252=CARTESIAN_POINT ( 'NONE',  ( -90.00000000000000000, -17.32050807568877815, -4.999999999999997335 ) ) ;
#2254=LINE ( 'NONE', #103, #397 ) ;
#2258=VECTOR ( 'NONE', #2782, 999.9999999999998863 ) ;
#2263=CIRCLE ( 'NONE', #2324, 22.50000000000000355 ) ;
#2268=SURFACE_STYLE_USAGE ( .BOTH. , #233 ) ;
#2272=ORIENTED_EDGE ( 'NONE', *, *, #1893, .T. ) ;
#2274=VECTOR ( 'NONE', #372, 999.9999999999998863 ) ;
#2277=DIRECTION ( 'NONE',  ( 0.000000000000000000, 0.000000000000000000, 1.000000000000000000 ) ) ;
#2286=ORIENTED_EDGE ( 'NONE', *, *, #2231, .T. ) ;
#2295=ORIENTED_EDGE ( 'NONE', *, *, #1284, .T. ) ;
#2296=CARTESIAN_POINT ( 'NONE',  ( -80.00000000000000000, 0.000000000000000000, 0.000000000000000000 ) ) ;
#2300=CARTESIAN_POINT ( 'NONE',  ( -70.00000000000000000, 0.000000000000000000, -30.00000000000000000 ) ) ;
#2304=DIRECTION ( 'NONE',  ( 0.000000000000000000, 0.000000000000000000, -1.000000000000000000 ) ) ;
#2309=VERTEX_POINT ( 'NONE', #1764 ) ;
#2314=DIRECTION ( 'NONE',  ( -1.000000000000000000, 0.000000000000000000, 0.000000000000000000 ) ) ;
#2324=AXIS2_PLACEMENT_3D ( 'NONE', #731, #2227, #64 ) ;
#2326=EDGE_CURVE ( 'NONE', #1234, #1799, #379, .T. ) ;
#2328=CARTESIAN_POINT ( 'NONE',  ( -4.500000000000000888, 0.000000000000000000, -24.00000000000000000 ) ) ;
#2329=EDGE_LOOP ( 'NONE', ( #2982, #3344, #411, #1398, #3109, #3779 ) ) ;
#2332=ORIENTED_EDGE ( 'NONE', *, *, #162, .T. ) ;
#2349=DIRECTION ( 'NONE',  ( 0.000000000000000000, 0.000000000000000000, 1.000000000000000000 ) ) ;
#2352=DIRECTION ( 'NONE',  ( 0.000000000000000000, 0.000000000000000000, 1.000000000000000000 ) ) ;
#2359=EDGE_CURVE ( 'NONE', #1737, #3824, #2441, .T. ) ;
#2367=ORIENTED_EDGE ( 'NONE', *, *, #1949, .F. ) ;
#2369=VERTEX_POINT ( 'NONE', #296 ) ;
#2386=AXIS2_PLACEMENT_3D ( 'NONE', #1870, #2478, #3127 ) ;
#2397=ORIENTED_EDGE ( 'NONE', *, *, #162, .F. ) ;
#2399=CARTESIAN_POINT ( 'NONE',  ( -90.00000000000000000, 0.000000000000000000, -30.00001199999999812 ) ) ;
#2412=FACE_OUTER_BOUND ( 'NONE', #2958, .T. ) ;
#2415=DIRECTION ( 'NONE',  ( -0.000000000000000000, 0.000000000000000000, 1.000000000000000000 ) ) ;
#2417=DIRECTION ( 'NONE',  ( -1.000000000000000000, 0.000000000000000000, 0.000000000000000000 ) ) ;
#2418=FACE_OUTER_BOUND ( 'NONE', #563, .T. ) ;
#2419=ORIENTED_EDGE ( 'NONE', *, *, #1126, .T. ) ;
#2422=VERTEX_POINT ( 'NONE', #2699 ) ;
#2441=CIRCLE ( 'NONE', #1441, 30.00000000000000000 ) ;
#2448=CARTESIAN_POINT ( 'NONE',  ( 0.000000000000000000, 0.000000000000000000, 0.000000000000000000 ) ) ;
#2452=AXIS2_PLACEMENT_3D ( 'NONE', #87, #1562, #2812 ) ;
#2454=FACE_OUTER_BOUND ( 'NONE', #1869, .T. ) ;
#2463=CARTESIAN_POINT ( 'NONE',  ( -80.00000000000000000, 0.000000000000000000, 23.28427124746188781 ) ) ;
#2465=PLANE ( 'NONE',  #2452 ) ;
#2470=FACE_BOUND ( 'NONE', #3831, .T. ) ;
#2478=DIRECTION ( 'NONE',  ( 0.000000000000000000, 0.000000000000000000, 1.000000000000000000 ) ) ;
#2487=CARTESIAN_POINT ( 'NONE',  ( 4.499999999999993783, 5.510910596163083639E-16, -30.00000000000000000 ) ) ;
#2490=DIRECTION ( 'NONE',  ( 1.000000000000000000, 0.000000000000000000, 0.000000000000000000 ) ) ;
#2494=ORIENTED_EDGE ( 'NONE', *, *, #3796, .T. ) ;
#2499=EDGE_CURVE ( 'NONE', #261, #1799, #914, .T. ) ;
#2513=CARTESIAN_POINT ( 'NONE',  ( 0.000000000000000000, 0.000000000000000000, 0.000000000000000000 ) ) ;
#2516=CIRCLE ( 'NONE', #332, 20.00000000000000000 ) ;
#2527=EDGE_LOOP ( 'NONE', ( #3103, #1127 ) ) ;
#2539=ADVANCED_FACE ( 'NONE', ( #3684, #425 ), #769, .T. ) ;
#2563=CARTESIAN_POINT ( 'NONE',  ( 0.000000000000000000, 0.000000000000000000, -24.00000000000000000 ) ) ;
#2564=FACE_OUTER_BOUND ( 'NONE', #2566, .T. ) ;
#2566=EDGE_LOOP ( 'NONE', ( #1967, #3632, #2419, #3724 ) ) ;
#2568=DIRECTION ( 'NONE',  ( 0.000000000000000000, -0.000000000000000000, -1.000000000000000000 ) ) ;
#2575=ORIENTED_EDGE ( 'NONE', *, *, #3359, .T. ) ;
#2576=ORIENTED_EDGE ( 'NONE', *, *, #3273, .F. ) ;
#2588=CARTESIAN_POINT ( 'NONE',  ( 2.000000000000001776, 2.449293598294708880E-16, -24.00000000000000000 ) ) ;
#2589=DIRECTION ( 'NONE',  ( -1.000000000000000000, 0.000000000000000000, 0.000000000000000000 ) ) ;
#2591=ADVANCED_FACE ( 'NONE', ( #3664 ), #116, .F. ) ;
#2594=( NAMED_UNIT ( * ) SI_UNIT ( $, .STERADIAN. ) SOLID_ANGLE_UNIT ( ) );
#2595=VERTEX_POINT ( 'NONE', #3111 ) ;
#2600=EDGE_LOOP ( 'NONE', ( #1767, #406, #927, #630 ) ) ;
#2605=CYLINDRICAL_SURFACE ( 'NONE', #2748, 2.000000000000001776 ) ;
#2609=DIRECTION ( 'NONE',  ( 0.000000000000000000, 0.000000000000000000, 1.000000000000000000 ) ) ;
#2612=EDGE_CURVE ( 'NONE', #2422, #758, #1310, .T. ) ;
#2621=AXIS2_PLACEMENT_3D ( 'NONE', #3424, #2568, #3720 ) ;
#2642=DIRECTION ( 'NONE',  ( 1.000000000000000000, 0.000000000000000000, -0.000000000000000000 ) ) ;
#2647=DIRECTION ( 'NONE',  ( -0.000000000000000000, 0.000000000000000000, 1.000000000000000000 ) ) ;
#2648=DIRECTION ( 'NONE',  ( -1.000000000000000000, 0.000000000000000000, 0.000000000000000000 ) ) ;
#2652=LINE ( 'NONE', #1286, #3516 ) ;
#2653=AXIS2_PLACEMENT_3D ( 'NONE', #1769, #2960, #285 ) ;
#2657=ORIENTED_EDGE ( 'NONE', *, *, #3556, .T. ) ;
#2662=DIRECTION ( 'NONE',  ( 0.000000000000000000, 0.000000000000000000, -1.000000000000000000 ) ) ;
#2663=DIRECTION ( 'NONE',  ( -0.000000000000000000, 0.000000000000000000, 1.000000000000000000 ) ) ;
#2667=CARTESIAN_POINT ( 'NONE',  ( -85.00000000000000000, 0.000000000000000000, 0.000000000000000000 ) ) ;
#2671=ORIENTED_EDGE ( 'NONE', *, *, #2231, .F. ) ;
#2672=DIRECTION ( 'NONE',  ( -0.000000000000000000, -0.000000000000000000, -1.000000000000000000 ) ) ;
#2677=ORIENTED_EDGE ( 'NONE', *, *, #26, .F. ) ;
#2688=PLANE ( 'NONE',  #2833 ) ;
#2693=ORIENTED_EDGE ( 'NONE', *, *, #1213, .T. ) ;
#2699=CARTESIAN_POINT ( 'NONE',  ( -3.749999999999998224, -29.76470224947664533, 0.000000000000000000 ) ) ;
#2700=AXIS2_PLACEMENT_3D ( 'NONE', #85, #3096, #452 ) ;
#2702=ORIENTED_EDGE ( 'NONE', *, *, #3443, .F. ) ;
#2704=FACE_BOUND ( 'NONE', #1772, .T. ) ;
#2710=( GEOMETRIC_REPRESENTATION_CONTEXT ( 3 ) GLOBAL_UNCERTAINTY_ASSIGNED_CONTEXT ( ( #3435 ) ) GLOBAL_UNIT_ASSIGNED_CONTEXT ( ( #3763, #3177, #2594 ) ) REPRESENTATION_CONTEXT ( 'NONE', 'WORKASPACE' ) );
#2711=VECTOR ( 'NONE', #1935, 1000.000000000000000 ) ;
#2717=ORIENTED_EDGE ( 'NONE', *, *, #1009, .T. ) ;
#2723=VERTEX_POINT ( 'NONE', #2134 ) ;
#2727=PRODUCT_DEFINITION_CONTEXT ( 'detailed design', #1375, 'design' ) ;
#2728=CARTESIAN_POINT ( 'NONE',  ( 0.000000000000000000, 0.000000000000000000, -24.00000000000000000 ) ) ;
#2733=DIRECTION ( 'NONE',  ( -0.000000000000000000, -0.000000000000000000, -1.000000000000000000 ) ) ;
#2741=CARTESIAN_POINT ( 'NONE',  ( -4.499999999999997335, 0.000000000000000000, -30.00000000000000000 ) ) ;
#2748=AXIS2_PLACEMENT_3D ( 'NONE', #838, #2061, #2648 ) ;
#2751=ORIENTED_EDGE ( 'NONE', *, *, #1949, .T. ) ;
#2762=DIRECTION ( 'NONE',  ( -1.000000000000000000, 0.000000000000000000, 0.000000000000000000 ) ) ;
#2764=AXIS2_PLACEMENT_3D ( 'NONE', #3653, #394, #3668 ) ;
#2766=CIRCLE ( 'NONE', #1217, 4.499999999999993783 ) ;
#2769=CARTESIAN_POINT ( 'NONE',  ( -82.50000000000000000, 19.84313483298442193, 0.000000000000000000 ) ) ;
#2770=VECTOR ( 'NONE', #962, 1000.000000000000000 ) ;
#2772=ORIENTED_EDGE ( 'NONE', *, *, #3326, .F. ) ;
#2781=EDGE_LOOP ( 'NONE', ( #850, #2079, #1976, #2074 ) ) ;
#2782=DIRECTION ( 'NONE',  ( 0.9921567416492215186, 0.1250000000000001665, 0.000000000000000000 ) ) ;
#2788=VERTEX_POINT ( 'NONE', #2667 ) ;
#2796=DIRECTION ( 'NONE',  ( -0.000000000000000000, -1.000000000000000000, -0.000000000000000000 ) ) ;
#2799=EDGE_CURVE ( 'NONE', #3418, #52, #2959, .T. ) ;
#2801=CARTESIAN_POINT ( 'NONE',  ( -3.749999999999998224, 29.76470224947664533, 0.000000000000000000 ) ) ;
#2802=DIRECTION ( 'NONE',  ( -0.9219985364506716463, 0.3871933609746164295, 0.000000000000000000 ) ) ;
#2809=AXIS2_PLACEMENT_3D ( 'NONE', #1185, #1986, #3497 ) ;
#2812=DIRECTION ( 'NONE',  ( 1.000000000000000000, 0.000000000000000000, 0.000000000000000000 ) ) ;
#2817=CIRCLE ( 'NONE', #3314, 1.325000000000000622 ) ;
#2818=VECTOR ( 'NONE', #1644, 1000.000000000000000 ) ;
#2819=CARTESIAN_POINT ( 'NONE',  ( -70.00000000000000000, 0.000000000000000000, -30.00001199999999812 ) ) ;
#2829=DIRECTION ( 'NONE',  ( -1.000000000000000000, 0.000000000000000000, 0.000000000000000000 ) ) ;
#2830=ORIENTED_EDGE ( 'NONE', *, *, #26, .T. ) ;
#2833=AXIS2_PLACEMENT_3D ( 'NONE', #3288, #58, #641 ) ;
#2834=VECTOR ( 'NONE', #2041, 1000.000000000000000 ) ;
#2835=DIRECTION ( 'NONE',  ( -0.000000000000000000, -0.000000000000000000, -1.000000000000000000 ) ) ;
#2837=LINE ( 'NONE', #1282, #3145 ) ;
#2842=ORIENTED_EDGE ( 'NONE', *, *, #665, .T. ) ;
#2848=DIRECTION ( 'NONE',  ( -0.9219985364506716463, 0.3871933609746164295, -2.048578313426146660E-17 ) ) ;
#2861=FACE_OUTER_BOUND ( 'NONE', #531, .T. ) ;
#2863=DIRECTION ( 'NONE',  ( -0.000000000000000000, 0.000000000000000000, 1.000000000000000000 ) ) ;
#2872=EDGE_CURVE ( 'NONE', #2788, #757, #1311, .T. ) ;
#2873=ADVANCED_FACE ( 'NONE', ( #1332 ), #3379, .F. ) ;
#2880=AXIS2_PLACEMENT_3D ( 'NONE', #2018, #1377, #2043 ) ;
#2883=( LENGTH_UNIT ( ) NAMED_UNIT ( * ) SI_UNIT ( .MILLI., .METRE. ) );
#2885=EDGE_LOOP ( 'NONE', ( #301, #307 ) ) ;
#2894=VECTOR ( 'NONE', #1317, 1000.000000000000000 ) ;
#2897=CIRCLE ( 'NONE', #3392, 30.00000000000000000 ) ;
#2903=ORIENTED_EDGE ( 'NONE', *, *, #566, .T. ) ;
#2905=CARTESIAN_POINT ( 'NONE',  ( 30.00000000000000000, 0.000000000000000000, -30.00000000000000000 ) ) ;
#2908=DIRECTION ( 'NONE',  ( -0.000000000000000000, -0.000000000000000000, -1.000000000000000000 ) ) ;
#2913=DIRECTION ( 'NONE',  ( 1.000000000000000000, 0.000000000000000000, 0.000000000000000000 ) ) ;
#2919=ADVANCED_FACE ( 'NONE', ( #142 ), #1872, .F. ) ;
#2921=EDGE_LOOP ( 'NONE', ( #2397, #3255, #3169, #3709 ) ) ;
#2925=EDGE_CURVE ( 'NONE', #1068, #143, #2137, .T. ) ;
#2931=EDGE_LOOP ( 'NONE', ( #3471, #3197, #2295, #1557 ) ) ;
#2932=CARTESIAN_POINT ( 'NONE',  ( -2.000000000000001776, 0.000000000000000000, -24.00000000000000000 ) ) ;
#2934=VERTEX_POINT ( 'NONE', #166 ) ;
#2936=CARTESIAN_POINT ( 'NONE',  ( -70.00000000000000000, 0.000000000000000000, -30.00000000000000000 ) ) ;
#2951=CARTESIAN_POINT ( 'NONE',  ( 30.00000000000000000, 0.000000000000000000, -30.00000000000000000 ) ) ;
#2956=COLOUR_RGB ( '',0.8941176470588234615, 0.8941176470588234615, 0.8941176470588234615 ) ;
#2958=EDGE_LOOP ( 'NONE', ( #2184, #115, #186, #3573, #2575 ) ) ;
#2959=LINE ( 'NONE', #2741, #141 ) ;
#2960=DIRECTION ( 'NONE',  ( 0.000000000000000000, 0.000000000000000000, -1.000000000000000000 ) ) ;
#2970=DIRECTION ( 'NONE',  ( 0.000000000000000000, 0.000000000000000000, 1.000000000000000000 ) ) ;
#2979=FACE_BOUND ( 'NONE', #1094, .T. ) ;
#2980=CARTESIAN_POINT ( 'NONE',  ( 0.000000000000000000, 0.000000000000000000, -30.00000000000000000 ) ) ;
#2982=ORIENTED_EDGE ( 'NONE', *, *, #164, .F. ) ;
#2984=CARTESIAN_POINT ( 'NONE',  ( -80.00000000000000000, 0.000000000000000000, 0.000000000000000000 ) ) ;
#2988=EDGE_LOOP ( 'NONE', ( #1014, #2332, #3123, #1726 ) ) ;
#2989=EDGE_CURVE ( 'NONE', #3050, #192, #3448, .T. ) ;
#2991=ORIENTED_EDGE ( 'NONE', *, *, #3159, .F. ) ;
#2993=VERTEX_POINT ( 'NONE', #2252 ) ;
#2995=LINE ( 'NONE', #918, #3271 ) ;
#2996=CYLINDRICAL_SURFACE ( 'NONE', #952, 2.000000000000001776 ) ;
#3001=CYLINDRICAL_SURFACE ( 'NONE', #1496, 30.00000000000000000 ) ;
#3004=CYLINDRICAL_SURFACE ( 'NONE', #3624, 30.00000000000000000 ) ;
#3019=AXIS2_PLACEMENT_3D ( 'NONE', #22, #2415, #3304 ) ;
#3020=AXIS2_PLACEMENT_3D ( 'NONE', #1851, #3660, #363 ) ;
#3041=DIRECTION ( 'NONE',  ( -0.000000000000000000, 0.000000000000000000, 1.000000000000000000 ) ) ;
#3043=CARTESIAN_POINT ( 'NONE',  ( -3.749999999999998224, -29.76470224947664533, -30.00000000000000000 ) ) ;
#3047=CARTESIAN_POINT ( 'NONE',  ( -3.749999999999998224, 29.76470224947664533, -30.00000000000000000 ) ) ;
#3050=VERTEX_POINT ( 'NONE', #1979 ) ;
#3063=CYLINDRICAL_SURFACE ( 'NONE', #3020, 5.000000000000004441 ) ;
#3072=DIRECTION ( 'NONE',  ( -0.000000000000000000, -0.000000000000000000, -1.000000000000000000 ) ) ;
#3091=VERTEX_POINT ( 'NONE', #1686 ) ;
#3096=DIRECTION ( 'NONE',  ( -0.000000000000000000, -0.000000000000000000, -1.000000000000000000 ) ) ;
#3100=LINE ( 'NONE', #3692, #3377 ) ;
#3103=ORIENTED_EDGE ( 'NONE', *, *, #1893, .F. ) ;
#3107=FACE_OUTER_BOUND ( 'NONE', #3380, .T. ) ;
#3109=ORIENTED_EDGE ( 'NONE', *, *, #1213, .F. ) ;
#3111=CARTESIAN_POINT ( 'NONE',  ( -75.00000000000000000, 6.123233995736772199E-16, -4.999999999999997335 ) ) ;
#3113=LINE ( 'NONE', #1008, #971 ) ;
#3118=DIRECTION ( 'NONE',  ( 1.000000000000000000, 0.000000000000000000, 0.000000000000000000 ) ) ;
#3123=ORIENTED_EDGE ( 'NONE', *, *, #3765, .T. ) ;
#3127=DIRECTION ( 'NONE',  ( 1.000000000000000000, 0.000000000000000000, -0.000000000000000000 ) ) ;
#3132=VECTOR ( 'NONE', #1736, 1000.000000000000000 ) ;
#3135=CARTESIAN_POINT ( 'NONE',  ( 20.00000000000000000, 0.000000000000000000, -20.00000000000000000 ) ) ;
#3139=DIRECTION ( 'NONE',  ( 0.000000000000000000, 0.000000000000000000, 1.000000000000000000 ) ) ;
#3143=( NAMED_UNIT ( * ) PLANE_ANGLE_UNIT ( ) SI_UNIT ( $, .RADIAN. ) );
#3145=VECTOR ( 'NONE', #3381, 1000.000000000000000 ) ;
#3158=CARTESIAN_POINT ( 'NONE',  ( -70.00000000000000000, -21.41798680385620202, -4.999999999999997335 ) ) ;
#3159=EDGE_CURVE ( 'NONE', #3824, #2309, #945, .T. ) ;
#3169=ORIENTED_EDGE ( 'NONE', *, *, #2799, .T. ) ;
#3175=DIRECTION ( 'NONE',  ( 0.000000000000000000, 0.000000000000000000, 1.000000000000000000 ) ) ;
#3177=( NAMED_UNIT ( * ) PLANE_ANGLE_UNIT ( ) SI_UNIT ( $, .RADIAN. ) );
#3179=CARTESIAN_POINT ( 'NONE',  ( -70.00000000000000000, 0.000000000000000000, -30.00001199999999812 ) ) ;
#3188=CARTESIAN_POINT ( 'NONE',  ( -4.499999999999993783, 0.000000000000000000, -30.00000000000000000 ) ) ;
#3194=DIRECTION ( 'NONE',  ( 1.000000000000000000, 0.000000000000000000, 0.000000000000000000 ) ) ;
#3196=AXIS2_PLACEMENT_3D ( 'NONE', #390, #2277, #493 ) ;
#3197=ORIENTED_EDGE ( 'NONE', *, *, #2499, .F. ) ;
#3201=UNCERTAINTY_MEASURE_WITH_UNIT (LENGTH_MEASURE( 1.000000000000000082E-05 ), #2883, 'distance_accuracy_value', 'NONE');
#3205=CARTESIAN_POINT ( 'NONE',  ( -82.50000000000000000, 19.84313483298442193, -30.00000000000000000 ) ) ;
#3217=CARTESIAN_POINT ( 'NONE',  ( -2.000000000000001776, 0.000000000000000000, -30.00000000000000000 ) ) ;
#3224=EDGE_CURVE ( 'NONE', #2993, #573, #826, .T. ) ;
#3225=EDGE_LOOP ( 'NONE', ( #1469, #2196, #3745, #3647 ) ) ;
#3237=DIRECTION ( 'NONE',  ( -0.000000000000000000, -0.000000000000000000, 1.000000000000000000 ) ) ;
#3241=CARTESIAN_POINT ( 'NONE',  ( -20.74496707014011676, 8.711850621928869387, 0.000000000000000000 ) ) ;
#3246=CIRCLE ( 'NONE', #2809, 5.000000000000004441 ) ;
#3250=CIRCLE ( 'NONE', #894, 20.00000000000000355 ) ;
#3254=DIRECTION ( 'NONE',  ( 1.000000000000000000, 0.000000000000000000, 0.000000000000000000 ) ) ;
#3255=ORIENTED_EDGE ( 'NONE', *, *, #977, .F. ) ;
#3265=CARTESIAN_POINT ( 'NONE',  ( 0.000000000000000000, 0.000000000000000000, 0.000000000000000000 ) ) ;
#3271=VECTOR ( 'NONE', #2081, 1000.000000000000000 ) ;
#3273=EDGE_CURVE ( 'NONE', #671, #385, #2263, .T. ) ;
#3282=DIRECTION ( 'NONE',  ( 0.000000000000000000, 0.000000000000000000, 1.000000000000000000 ) ) ;
#3285=DIRECTION ( 'NONE',  ( 1.000000000000000000, 0.000000000000000000, 0.000000000000000000 ) ) ;
#3288=CARTESIAN_POINT ( 'NONE',  ( -3.750000000000001776, -29.76470224947664178, -30.00000000000000000 ) ) ;
#3289=FACE_OUTER_BOUND ( 'NONE', #242, .T. ) ;
#3292=EDGE_LOOP ( 'NONE', ( #1462, #1160 ) ) ;
#3293=ORIENTED_EDGE ( 'NONE', *, *, #977, .T. ) ;
#3303=VECTOR ( 'NONE', #434, 1000.000000000000000 ) ;
#3304=DIRECTION ( 'NONE',  ( 1.000000000000000000, 0.000000000000000000, 0.000000000000000000 ) ) ;
#3308=ADVANCED_FACE ( 'NONE', ( #2035 ), #849, .F. ) ;
#3312=CARTESIAN_POINT ( 'NONE',  ( -75.00000000000000000, 6.123233995736772199E-16, 0.001000000000000132727 ) ) ;
#3314=AXIS2_PLACEMENT_3D ( 'NONE', #2121, #1021, #2802 ) ;
#3318=EDGE_LOOP ( 'NONE', ( #1743, #1621, #2657, #180 ) ) ;
#3326=EDGE_CURVE ( 'NONE', #2993, #276, #1352, .T. ) ;
#3329=ADVANCED_FACE ( 'NONE', ( #446 ), #1682, .T. ) ;
#3331=DIRECTION ( 'NONE',  ( -0.000000000000000000, 0.000000000000000000, 1.000000000000000000 ) ) ;
#3336=DIRECTION ( 'NONE',  ( -0.000000000000000000, -0.000000000000000000, 1.000000000000000000 ) ) ;
#3341=CLOSED_SHELL ( 'NONE', ( #2919, #1988, #3308, #2230, #1406, #1746, #1663, #678, #361, #1436, #2591, #3542, #1929, #2539, #3717, #937, #389, #3329, #1667, #2873, #3722, #1887, #2238, #1140 ) ) ;
#3343=CARTESIAN_POINT ( 'NONE',  ( 0.000000000000000000, 0.000000000000000000, -24.00000000000000000 ) ) ;
#3344=ORIENTED_EDGE ( 'NONE', *, *, #517, .F. ) ;
#3346=LINE ( 'NONE', #1603, #88 ) ;
#3350=LINE ( 'NONE', #1850, #2770 ) ;
#3357=ORIENTED_EDGE ( 'NONE', *, *, #1284, .F. ) ;
#3359=EDGE_CURVE ( 'NONE', #3615, #758, #3250, .T. ) ;
#3373=ORIENTED_EDGE ( 'NONE', *, *, #3359, .F. ) ;
#3377=VECTOR ( 'NONE', #3735, 1000.000000000000000 ) ;
#3379=CYLINDRICAL_SURFACE ( 'NONE', #207, 9.999999999999994671 ) ;
#3380=EDGE_LOOP ( 'NONE', ( #2772, #1490, #2693, #3373, #36, #1747 ) ) ;
#3381=DIRECTION ( 'NONE',  ( 0.000000000000000000, 0.000000000000000000, 1.000000000000000000 ) ) ;
#3388=STYLED_ITEM ( 'NONE', ( #1974 ), #791 ) ;
#3391=LINE ( 'NONE', #3312, #1336 ) ;
#3392=AXIS2_PLACEMENT_3D ( 'NONE', #1102, #190, #803 ) ;
#3399=CIRCLE ( 'NONE', #2159, 2.000000000000001776 ) ;
#3402=FACE_BOUND ( 'NONE', #2527, .T. ) ;
#3418=VERTEX_POINT ( 'NONE', #2328 ) ;
#3424=CARTESIAN_POINT ( 'NONE',  ( -80.00000000000000000, 0.000000000000000000, 0.000000000000000000 ) ) ;
#3429=PRODUCT_DEFINITION_SHAPE ( 'NONE', 'NONE',  #1794 ) ;
#3431=CIRCLE ( 'NONE', #1752, 20.00000000000000355 ) ;
#3435=UNCERTAINTY_MEASURE_WITH_UNIT (LENGTH_MEASURE( 1.000000000000000082E-05 ), #3763, 'distance_accuracy_value', 'NONE');
#3437=ORIENTED_EDGE ( 'NONE', *, *, #1897, .T. ) ;
#3443=EDGE_CURVE ( 'NONE', #2072, #328, #3562, .T. ) ;
#3448=CIRCLE ( 'NONE', #3196, 2.000000000000001776 ) ;
#3453=MECHANICAL_DESIGN_GEOMETRIC_PRESENTATION_REPRESENTATION('',(#3388),#2710);
#3471=ORIENTED_EDGE ( 'NONE', *, *, #2326, .T. ) ;
#3475=DIRECTION ( 'NONE',  ( -1.000000000000000000, 0.000000000000000000, 0.000000000000000000 ) ) ;
#3483=ORIENTED_EDGE ( 'NONE', *, *, #517, .T. ) ;
#3494=AXIS2_PLACEMENT_3D ( 'NONE', #581, #1431, #1770 ) ;
#3497=DIRECTION ( 'NONE',  ( -1.000000000000000000, 0.000000000000000000, 0.000000000000000000 ) ) ;
#3513=CARTESIAN_POINT ( 'NONE',  ( 0.000000000000000000, 0.000000000000000000, 0.000000000000000000 ) ) ;
#3516=VECTOR ( 'NONE', #2796, 1000.000000000000000 ) ;
#3517=LINE ( 'NONE', #1447, #1879 ) ;
#3519=CIRCLE ( 'NONE', #598, 20.00000000000000000 ) ;
#3522=( NAMED_UNIT ( * ) SI_UNIT ( $, .STERADIAN. ) SOLID_ANGLE_UNIT ( ) );
#3532=EDGE_CURVE ( 'NONE', #2369, #2723, #2129, .T. ) ;
#3542=ADVANCED_FACE ( 'NONE', ( #2418 ), #3004, .T. ) ;
#3556=EDGE_CURVE ( 'NONE', #192, #1068, #3604, .T. ) ;
#3558=CIRCLE ( 'NONE', #1700, 20.00000000000000000 ) ;
#3562=CIRCLE ( 'NONE', #2190, 20.00000000000000000 ) ;
#3568=CARTESIAN_POINT ( 'NONE',  ( 0.000000000000000000, 0.000000000000000000, -30.00000000000000000 ) ) ;
#3572=DIRECTION ( 'NONE',  ( -1.000000000000000000, 1.776356839400250070E-15, 0.000000000000000000 ) ) ;
#3573=ORIENTED_EDGE ( 'NONE', *, *, #516, .F. ) ;
#3604=LINE ( 'NONE', #3217, #3132 ) ;
#3615=VERTEX_POINT ( 'NONE', #2769 ) ;
#3621=CARTESIAN_POINT ( 'NONE',  ( 20.74496707014011676, -8.711850621928872940, 0.000000000000000000 ) ) ;
#3624=AXIS2_PLACEMENT_3D ( 'NONE', #3568, #2970, #1233 ) ;
#3630=AXIS2_PLACEMENT_3D ( 'NONE', #3343, #3072, #369 ) ;
#3632=ORIENTED_EDGE ( 'NONE', *, *, #1777, .T. ) ;
#3639=DIRECTION ( 'NONE',  ( 0.000000000000000000, -0.000000000000000000, -1.000000000000000000 ) ) ;
#3643=PRODUCT ( 'shuttle unit', 'shuttle unit', '', ( #1948 ) ) ;
#3644=EDGE_CURVE ( 'NONE', #385, #2723, #2817, .T. ) ;
#3647=ORIENTED_EDGE ( 'NONE', *, *, #1121, .T. ) ;
#3653=CARTESIAN_POINT ( 'NONE',  ( 21.96661513093725659, -9.224881825220240472, -2.544523588129261943E-16 ) ) ;
#3656=FACE_OUTER_BOUND ( 'NONE', #655, .T. ) ;
#3660=DIRECTION ( 'NONE',  ( -0.000000000000000000, -0.000000000000000000, -1.000000000000000000 ) ) ;
#3663=ORIENTED_EDGE ( 'NONE', *, *, #2989, .F. ) ;
#3664=FACE_OUTER_BOUND ( 'NONE', #3225, .T. ) ;
#3666=VERTEX_POINT ( 'NONE', #3047 ) ;
#3667=CARTESIAN_POINT ( 'NONE',  ( -75.00000000000000000, 6.123233995736772199E-16, 0.000000000000000000 ) ) ;
#3668=DIRECTION ( 'NONE',  ( 0.9219985364506716463, -0.3871933609746164295, 0.000000000000000000 ) ) ;
#3673=LINE ( 'NONE', #1882, #2258 ) ;
#3678=EDGE_CURVE ( 'NONE', #52, #1782, #1323, .T. ) ;
#3684=FACE_BOUND ( 'NONE', #1687, .T. ) ;
#3692=CARTESIAN_POINT ( 'NONE',  ( 2.000000000000001776, 2.449293598294708880E-16, -30.00000000000000000 ) ) ;
#3704=CYLINDRICAL_SURFACE ( 'NONE', #528, 20.00000000000000000 ) ;
#3709=ORIENTED_EDGE ( 'NONE', *, *, #3678, .T. ) ;
#3717=ADVANCED_FACE ( 'NONE', ( #2454 ), #3704, .F. ) ;
#3720=DIRECTION ( 'NONE',  ( 1.000000000000000000, 0.000000000000000000, 0.000000000000000000 ) ) ;
#3722=ADVANCED_FACE ( 'NONE', ( #1595 ), #3063, .F. ) ;
#3724=ORIENTED_EDGE ( 'NONE', *, *, #304, .F. ) ;
#3725=DIRECTION ( 'NONE',  ( -0.000000000000000000, -0.000000000000000000, -1.000000000000000000 ) ) ;
#3728=EDGE_CURVE ( 'NONE', #1003, #2595, #3391, .T. ) ;
#3735=DIRECTION ( 'NONE',  ( -0.000000000000000000, -0.000000000000000000, -1.000000000000000000 ) ) ;
#3737=EDGE_CURVE ( 'NONE', #2422, #2309, #1962, .T. ) ;
#3738=ORIENTED_EDGE ( 'NONE', *, *, #854, .T. ) ;
#3743=DIRECTION ( 'NONE',  ( -1.795453617517838654E-17, 1.015442787603507153E-17, 1.000000000000000000 ) ) ;
#3745=ORIENTED_EDGE ( 'NONE', *, *, #1820, .F. ) ;
#3746=CIRCLE ( 'NONE', #2186, 5.000000000000004441 ) ;
#3747=CARTESIAN_POINT ( 'NONE',  ( 0.000000000000000000, 0.000000000000000000, -20.00000000000000000 ) ) ;
#3763=( LENGTH_UNIT ( ) NAMED_UNIT ( * ) SI_UNIT ( .MILLI., .METRE. ) );
#3764=AXIS2_PLACEMENT_3D ( 'NONE', #3265, #2647, #3285 ) ;
#3765=EDGE_CURVE ( 'NONE', #1782, #52, #2766, .T. ) ;
#3777=PLANE ( 'NONE',  #1199 ) ;
#3779=ORIENTED_EDGE ( 'NONE', *, *, #1009, .F. ) ;
#3780=LINE ( 'NONE', #1675, #1781 ) ;
#3794=CARTESIAN_POINT ( 'NONE',  ( 0.000000000000000000, 0.000000000000000000, 0.000000000000000000 ) ) ;
#3796=EDGE_CURVE ( 'NONE', #328, #2072, #2516, .T. ) ;
#3809=CARTESIAN_POINT ( 'NONE',  ( -2.000000000000001776, 0.000000000000000000, -20.00000000000000000 ) ) ;
#3824=VERTEX_POINT ( 'NONE', #2905 ) ;
#3831=EDGE_LOOP ( 'NONE', ( #2040, #1993 ) ) ;
#3854=COLOUR_RGB('Light Blue',0.38,0.62,0.78);
#3855=FILL_AREA_STYLE_COLOUR('',#3854);
#3856=FILL_AREA_STYLE('',(#3855));
#3857=SURFACE_STYLE_FILL_AREA(#3856);
#3858=SURFACE_SIDE_STYLE('',(#3857));
#3859=SURFACE_STYLE_USAGE(.BOTH.,#3858);
#3860=PRESENTATION_STYLE_ASSIGNMENT((#3859));
ENDSEC;
END-ISO-10303-21;
